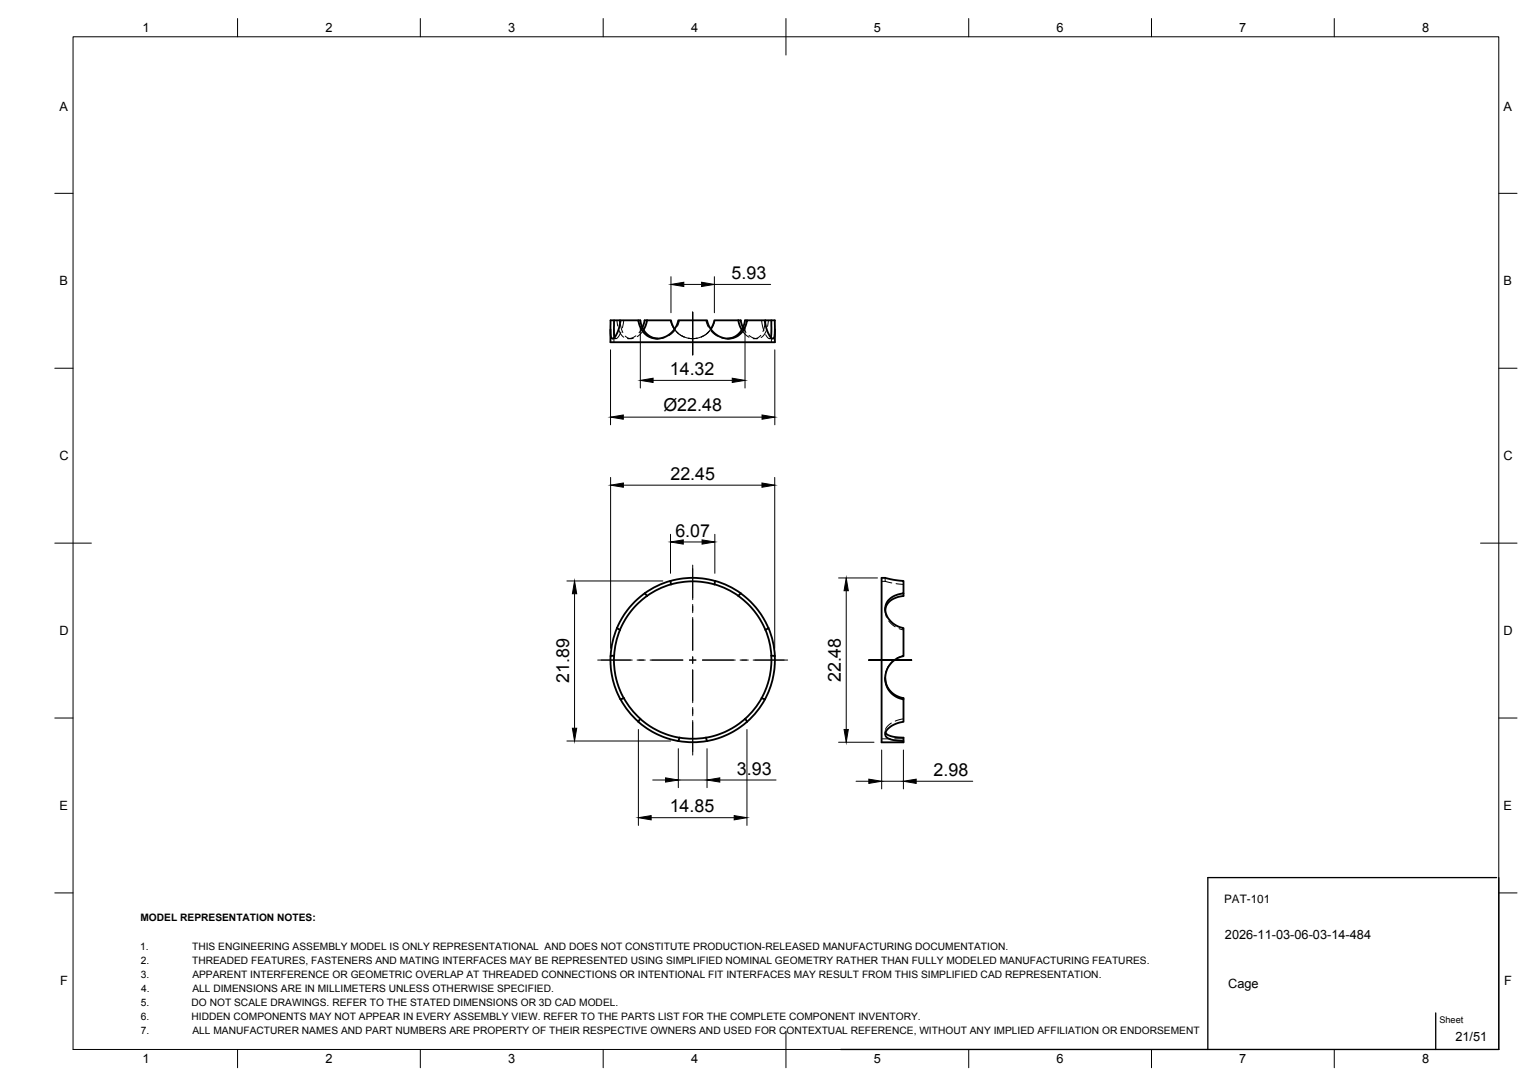
ISO-10303-21;
HEADER;
/* Generated by software containing ST-Developer
 * from STEP Tools, Inc. (www.steptools.com) 
 */

FILE_DESCRIPTION(
/* description */ ('Spur gear reduction stage 2-1 on bearing plates'),
/* implementation_level */ '2;1');

FILE_NAME(
/* name */ 'Cage.step',
/* time_stamp */ '2026-10-28T03:22:07-07:00',
/* author */ (''),
/* organization */ (''),
/* preprocessor_version */ 'ST-DEVELOPER v20.2',
/* originating_system */ 'Autodesk Translation Framework v15.17.0.0',
/* authorisation */ '');

FILE_SCHEMA (('AUTOMOTIVE_DESIGN { 1 0 10303 214 3 1 1 }'));
ENDSEC;

DATA;
#10=MECHANICAL_DESIGN_GEOMETRIC_PRESENTATION_REPRESENTATION('',(#969),#53909);
#667=B_SPLINE_CURVE_WITH_KNOTS('',3,(#16802,#16803,#16804,#16805,#16806,
#16807,#16808,#16809,#16810,#16811,#16812,#16813,#16814,#16815,#16816,#16817,
#16818,#16819,#16820,#16821,#16822,#16823),.UNSPECIFIED.,.F.,.F.,(4,2,2,
2,2,2,2,2,2,2,4),(0.0591825211272536,0.157966726598481,0.236950089897721,
0.315933453196962,0.391576304923761,0.46721915665056,0.54286200837736,0.618504860104159,
0.697488223403399,0.77647158670264,0.875255792173867),.UNSPECIFIED.);
#668=B_SPLINE_CURVE_WITH_KNOTS('',3,(#16827,#16828,#16829,#16830,#16831,
#16832,#16833,#16834,#16835,#16836,#16837,#16838,#16839,#16840,#16841,#16842,
#16843,#16844,#16845,#16846,#16847,#16848),.UNSPECIFIED.,.F.,.F.,(4,2,2,
2,2,2,2,2,2,2,4),(0.0581119756758434,0.106553146291161,0.213106292582322,
0.30849933801665,0.386091982889075,0.4636846277615,0.541277272633925,0.61886991750635,
0.714262962940678,0.820816109231839,0.869257279847157),.UNSPECIFIED.);
#669=B_SPLINE_CURVE_WITH_KNOTS('',3,(#16854,#16855,#16856,#16857,#16858,
#16859,#16860,#16861,#16862,#16863,#16864,#16865,#16866,#16867,#16868,#16869,
#16870,#16871,#16872,#16873,#16874,#16875),.UNSPECIFIED.,.F.,.F.,(4,2,2,
2,2,2,2,2,2,2,4),(0.0581119756758434,0.106553146291161,0.213106292582322,
0.30849933801665,0.386091982889075,0.4636846277615,0.541277272633925,0.61886991750635,
0.714262962940679,0.820816109231839,0.869257279847157),.UNSPECIFIED.);
#670=B_SPLINE_CURVE_WITH_KNOTS('',3,(#16879,#16880,#16881,#16882,#16883,
#16884,#16885,#16886,#16887,#16888,#16889,#16890,#16891,#16892,#16893,#16894,
#16895,#16896,#16897,#16898,#16899,#16900),.UNSPECIFIED.,.F.,.F.,(4,2,2,
2,2,2,2,2,2,2,4),(0.0581119756758433,0.106553146291161,0.213106292582322,
0.308499338016649,0.386091982889075,0.4636846277615,0.541277272633925,0.61886991750635,
0.714262962940678,0.820816109231839,0.869257279847157),.UNSPECIFIED.);
#671=B_SPLINE_CURVE_WITH_KNOTS('',3,(#16909,#16910,#16911,#16912,#16913,
#16914,#16915,#16916,#16917,#16918,#16919,#16920,#16921,#16922,#16923,#16924,
#16925,#16926,#16927,#16928,#16929,#16930),.UNSPECIFIED.,.F.,.F.,(4,2,2,
2,2,2,2,2,2,2,4),(0.0581119756758433,0.106553146291161,0.213106292582322,
0.30849933801665,0.386091982889075,0.4636846277615,0.541277272633925,0.61886991750635,
0.714262962940678,0.820816109231839,0.869257279847157),.UNSPECIFIED.);
#672=B_SPLINE_CURVE_WITH_KNOTS('',3,(#16934,#16935,#16936,#16937,#16938,
#16939,#16940,#16941,#16942,#16943,#16944,#16945,#16946,#16947,#16948,#16949,
#16950,#16951,#16952,#16953,#16954,#16955),.UNSPECIFIED.,.F.,.F.,(4,2,2,
2,2,2,2,2,2,2,4),(0.0581119756758434,0.106553146291161,0.213106292582322,
0.30849933801665,0.386091982889075,0.4636846277615,0.541277272633925,0.61886991750635,
0.714262962940678,0.820816109231839,0.869257279847157),.UNSPECIFIED.);
#673=B_SPLINE_CURVE_WITH_KNOTS('',3,(#16959,#16960,#16961,#16962,#16963,
#16964,#16965,#16966,#16967,#16968,#16969,#16970,#16971,#16972,#16973,#16974,
#16975,#16976,#16977,#16978,#16979,#16980),.UNSPECIFIED.,.F.,.F.,(4,2,2,
2,2,2,2,2,2,2,4),(0.0581119756758434,0.106553146291161,0.213106292582322,
0.30849933801665,0.386091982889075,0.4636846277615,0.541277272633925,0.61886991750635,
0.714262962940678,0.820816109231839,0.869257279847157),.UNSPECIFIED.);
#674=B_SPLINE_CURVE_WITH_KNOTS('',3,(#16984,#16985,#16986,#16987,#16988,
#16989,#16990,#16991,#16992,#16993,#16994,#16995,#16996,#16997,#16998,#16999,
#17000,#17001,#17002,#17003,#17004,#17005),.UNSPECIFIED.,.F.,.F.,(4,2,2,
2,2,2,2,2,2,2,4),(0.0581119756758433,0.106553146291161,0.213106292582322,
0.30849933801665,0.386091982889075,0.4636846277615,0.541277272633925,0.61886991750635,
0.714262962940678,0.820816109231839,0.869257279847157),.UNSPECIFIED.);
#675=B_SPLINE_CURVE_WITH_KNOTS('',3,(#17013,#17014,#17015,#17016,#17017,
#17018,#17019,#17020,#17021,#17022,#17023,#17024,#17025,#17026,#17027,#17028,
#17029,#17030,#17031,#17032,#17033,#17034),.UNSPECIFIED.,.F.,.F.,(4,2,2,
2,2,2,2,2,2,2,4),(0.0591825211272536,0.157966726598481,0.236950089897721,
0.315933453196962,0.391576304923761,0.467219156650561,0.54286200837736,
0.618504860104159,0.697488223403399,0.77647158670264,0.875255792173867),
 .UNSPECIFIED.);
#676=B_SPLINE_CURVE_WITH_KNOTS('',3,(#17042,#17043,#17044,#17045,#17046,
#17047,#17048,#17049,#17050,#17051,#17052,#17053,#17054,#17055,#17056,#17057,
#17058,#17059,#17060,#17061,#17062,#17063),.UNSPECIFIED.,.F.,.F.,(4,2,2,
2,2,2,2,2,2,2,4),(0.0591825211272536,0.157966726598481,0.236950089897722,
0.315933453196962,0.391576304923761,0.467219156650561,0.54286200837736,
0.618504860104159,0.697488223403399,0.77647158670264,0.875255792173867),
 .UNSPECIFIED.);
#677=B_SPLINE_CURVE_WITH_KNOTS('',3,(#17073,#17074,#17075,#17076,#17077,
#17078,#17079,#17080,#17081,#17082,#17083,#17084,#17085,#17086,#17087,#17088,
#17089,#17090,#17091,#17092,#17093,#17094),.UNSPECIFIED.,.F.,.F.,(4,2,2,
2,2,2,2,2,2,2,4),(0.0591825211272536,0.157966726598481,0.236950089897721,
0.315933453196962,0.391576304923761,0.46721915665056,0.54286200837736,0.618504860104159,
0.697488223403399,0.77647158670264,0.875255792173867),.UNSPECIFIED.);
#678=B_SPLINE_CURVE_WITH_KNOTS('',3,(#17102,#17103,#17104,#17105,#17106,
#17107,#17108,#17109,#17110,#17111,#17112,#17113,#17114,#17115,#17116,#17117,
#17118,#17119,#17120,#17121,#17122,#17123),.UNSPECIFIED.,.F.,.F.,(4,2,2,
2,2,2,2,2,2,2,4),(0.0591825211272536,0.157966726598481,0.236950089897721,
0.315933453196962,0.391576304923761,0.46721915665056,0.542862008377359,
0.618504860104159,0.697488223403399,0.776471586702639,0.875255792173867),
 .UNSPECIFIED.);
#679=B_SPLINE_CURVE_WITH_KNOTS('',3,(#17131,#17132,#17133,#17134,#17135,
#17136,#17137,#17138,#17139,#17140,#17141,#17142,#17143,#17144,#17145,#17146,
#17147,#17148,#17149,#17150,#17151,#17152),.UNSPECIFIED.,.F.,.F.,(4,2,2,
2,2,2,2,2,2,2,4),(0.0591825211272536,0.157966726598481,0.236950089897721,
0.315933453196962,0.391576304923761,0.46721915665056,0.54286200837736,0.618504860104159,
0.697488223403399,0.77647158670264,0.875255792173867),.UNSPECIFIED.);
#680=B_SPLINE_CURVE_WITH_KNOTS('',3,(#17161,#17162,#17163,#17164,#17165,
#17166,#17167,#17168,#17169,#17170,#17171,#17172,#17173,#17174,#17175,#17176,
#17177,#17178,#17179,#17180,#17181,#17182),.UNSPECIFIED.,.F.,.F.,(4,2,2,
2,2,2,2,2,2,2,4),(0.0591825211272536,0.157966726598481,0.236950089897721,
0.315933453196962,0.391576304923761,0.46721915665056,0.542862008377359,
0.618504860104159,0.697488223403399,0.776471586702639,0.875255792173867),
 .UNSPECIFIED.);
#802=SPHERICAL_SURFACE('',#12210,0.309556);
#803=SPHERICAL_SURFACE('',#12226,0.309556);
#804=SPHERICAL_SURFACE('',#12231,0.309556);
#805=SPHERICAL_SURFACE('',#12237,0.309556);
#806=SPHERICAL_SURFACE('',#12242,0.309556);
#807=SPHERICAL_SURFACE('',#12247,0.309556);
#808=SPHERICAL_SURFACE('',#12255,0.309556);
#877=SHAPE_REPRESENTATION_RELATIONSHIP('SRR','None',#54105,#920);
#920=ADVANCED_BREP_SHAPE_REPRESENTATION('',(#1025),#53879);
#969=STYLED_ITEM('',(#54397),#1025);
#1025=MANIFOLD_SOLID_BREP('Continuous crown cage',#11295);
#1182=FACE_BOUND('',#2476,.T.);
#1318=PLANE('',#12223);
#1319=PLANE('',#12228);
#1320=PLANE('',#12233);
#1321=PLANE('',#12239);
#1322=PLANE('',#12244);
#1323=PLANE('',#12253);
#1324=PLANE('',#12257);
#1325=PLANE('',#12258);
#1690=FACE_OUTER_BOUND('',#2460,.T.);
#1691=FACE_OUTER_BOUND('',#2461,.T.);
#1692=FACE_OUTER_BOUND('',#2462,.T.);
#1693=FACE_OUTER_BOUND('',#2463,.T.);
#1694=FACE_OUTER_BOUND('',#2464,.T.);
#1695=FACE_OUTER_BOUND('',#2465,.T.);
#1696=FACE_OUTER_BOUND('',#2466,.T.);
#1697=FACE_OUTER_BOUND('',#2467,.T.);
#1698=FACE_OUTER_BOUND('',#2468,.T.);
#1699=FACE_OUTER_BOUND('',#2469,.T.);
#1700=FACE_OUTER_BOUND('',#2470,.T.);
#1701=FACE_OUTER_BOUND('',#2471,.T.);
#1702=FACE_OUTER_BOUND('',#2472,.T.);
#1703=FACE_OUTER_BOUND('',#2473,.T.);
#1704=FACE_OUTER_BOUND('',#2474,.T.);
#1705=FACE_OUTER_BOUND('',#2475,.T.);
#1706=FACE_OUTER_BOUND('',#2477,.T.);
#2460=EDGE_LOOP('',(#8086,#8087,#8088,#8089));
#2461=EDGE_LOOP('',(#8090,#8091,#8092,#8093,#8094,#8095,#8096,#8097,#8098,
#8099,#8100,#8101,#8102,#8103,#8104,#8105,#8106,#8107));
#2462=EDGE_LOOP('',(#8108,#8109,#8110,#8111));
#2463=EDGE_LOOP('',(#8112,#8113,#8114,#8115));
#2464=EDGE_LOOP('',(#8116,#8117,#8118,#8119));
#2465=EDGE_LOOP('',(#8120,#8121,#8122,#8123));
#2466=EDGE_LOOP('',(#8124,#8125,#8126,#8127,#8128,#8129));
#2467=EDGE_LOOP('',(#8130,#8131,#8132,#8133));
#2468=EDGE_LOOP('',(#8134,#8135,#8136,#8137));
#2469=EDGE_LOOP('',(#8138,#8139,#8140,#8141));
#2470=EDGE_LOOP('',(#8142,#8143,#8144,#8145));
#2471=EDGE_LOOP('',(#8146,#8147,#8148,#8149));
#2472=EDGE_LOOP('',(#8150,#8151,#8152,#8153,#8154,#8155,#8156,#8157,#8158,
#8159,#8160,#8161,#8162,#8163,#8164,#8165,#8166,#8167));
#2473=EDGE_LOOP('',(#8168,#8169,#8170,#8171));
#2474=EDGE_LOOP('',(#8172,#8173,#8174,#8175));
#2475=EDGE_LOOP('',(#8176));
#2476=EDGE_LOOP('',(#8177));
#2477=EDGE_LOOP('',(#8178,#8179,#8180,#8181));
#3147=LINE('',#16904,#3788);
#3148=LINE('',#17157,#3789);
#3788=VECTOR('',#13974,1.123812);
#3789=VECTOR('',#14043,1.076188);
#4456=CIRCLE('',#12211,0.303778037777585);
#4457=CIRCLE('',#12212,0.303778037777585);
#4458=CIRCLE('',#12214,1.123812);
#4459=CIRCLE('',#12215,1.123812);
#4460=CIRCLE('',#12216,1.123812);
#4461=CIRCLE('',#12217,1.123812);
#4462=CIRCLE('',#12218,1.123812);
#4463=CIRCLE('',#12219,1.123812);
#4464=CIRCLE('',#12220,1.123812);
#4465=CIRCLE('',#12221,1.123812);
#4466=CIRCLE('',#12222,1.123812);
#4467=CIRCLE('',#12224,1.076188);
#4468=CIRCLE('',#12225,0.303778037777585);
#4469=CIRCLE('',#12227,0.303778037777585);
#4470=CIRCLE('',#12229,1.076188);
#4471=CIRCLE('',#12230,0.303778037777585);
#4472=CIRCLE('',#12232,0.303778037777585);
#4473=CIRCLE('',#12234,1.076188);
#4474=CIRCLE('',#12235,1.076188);
#4475=CIRCLE('',#12236,0.303778037777585);
#4476=CIRCLE('',#12238,0.303778037777585);
#4477=CIRCLE('',#12240,1.076188);
#4478=CIRCLE('',#12241,0.303778037777585);
#4479=CIRCLE('',#12243,0.303778037777585);
#4480=CIRCLE('',#12245,1.076188);
#4481=CIRCLE('',#12246,0.303778037777585);
#4482=CIRCLE('',#12248,0.303778037777585);
#4483=CIRCLE('',#12250,1.076188);
#4484=CIRCLE('',#12251,1.076188);
#4485=CIRCLE('',#12252,1.076188);
#4486=CIRCLE('',#12254,0.303778037777585);
#4487=CIRCLE('',#12256,0.303778037777585);
#5034=VERTEX_POINT('',#16800);
#5035=VERTEX_POINT('',#16801);
#5036=VERTEX_POINT('',#16824);
#5037=VERTEX_POINT('',#16826);
#5038=VERTEX_POINT('',#16851);
#5039=VERTEX_POINT('',#16853);
#5040=VERTEX_POINT('',#16876);
#5041=VERTEX_POINT('',#16878);
#5042=VERTEX_POINT('',#16901);
#5043=VERTEX_POINT('',#16903);
#5044=VERTEX_POINT('',#16906);
#5045=VERTEX_POINT('',#16908);
#5046=VERTEX_POINT('',#16931);
#5047=VERTEX_POINT('',#16933);
#5048=VERTEX_POINT('',#16956);
#5049=VERTEX_POINT('',#16958);
#5050=VERTEX_POINT('',#16981);
#5051=VERTEX_POINT('',#16983);
#5052=VERTEX_POINT('',#17008);
#5053=VERTEX_POINT('',#17012);
#5054=VERTEX_POINT('',#17037);
#5055=VERTEX_POINT('',#17041);
#5056=VERTEX_POINT('',#17066);
#5057=VERTEX_POINT('',#17068);
#5058=VERTEX_POINT('',#17072);
#5059=VERTEX_POINT('',#17097);
#5060=VERTEX_POINT('',#17101);
#5061=VERTEX_POINT('',#17126);
#5062=VERTEX_POINT('',#17130);
#5063=VERTEX_POINT('',#17155);
#5064=VERTEX_POINT('',#17158);
#5065=VERTEX_POINT('',#17160);
#6185=EDGE_CURVE('',#5034,#5035,#667,.T.);
#6186=EDGE_CURVE('',#5036,#5034,#4456,.T.);
#6187=EDGE_CURVE('',#5037,#5036,#668,.T.);
#6188=EDGE_CURVE('',#5035,#5037,#4457,.T.);
#6189=EDGE_CURVE('',#5038,#5036,#4458,.T.);
#6190=EDGE_CURVE('',#5038,#5039,#669,.T.);
#6191=EDGE_CURVE('',#5040,#5039,#4459,.T.);
#6192=EDGE_CURVE('',#5040,#5041,#670,.T.);
#6193=EDGE_CURVE('',#5042,#5041,#4460,.T.);
#6194=EDGE_CURVE('',#5042,#5043,#3147,.T.);
#6195=EDGE_CURVE('',#5043,#5043,#4461,.T.);
#6196=EDGE_CURVE('',#5044,#5042,#4462,.T.);
#6197=EDGE_CURVE('',#5044,#5045,#671,.T.);
#6198=EDGE_CURVE('',#5046,#5045,#4463,.T.);
#6199=EDGE_CURVE('',#5046,#5047,#672,.T.);
#6200=EDGE_CURVE('',#5048,#5047,#4464,.T.);
#6201=EDGE_CURVE('',#5048,#5049,#673,.T.);
#6202=EDGE_CURVE('',#5050,#5049,#4465,.T.);
#6203=EDGE_CURVE('',#5050,#5051,#674,.T.);
#6204=EDGE_CURVE('',#5037,#5051,#4466,.T.);
#6205=EDGE_CURVE('',#5034,#5052,#4467,.T.);
#6206=EDGE_CURVE('',#5052,#5038,#4468,.T.);
#6207=EDGE_CURVE('',#5053,#5052,#675,.T.);
#6208=EDGE_CURVE('',#5039,#5053,#4469,.T.);
#6209=EDGE_CURVE('',#5053,#5054,#4470,.T.);
#6210=EDGE_CURVE('',#5054,#5040,#4471,.T.);
#6211=EDGE_CURVE('',#5055,#5054,#676,.T.);
#6212=EDGE_CURVE('',#5041,#5055,#4472,.T.);
#6213=EDGE_CURVE('',#5055,#5056,#4473,.T.);
#6214=EDGE_CURVE('',#5056,#5057,#4474,.T.);
#6215=EDGE_CURVE('',#5057,#5044,#4475,.T.);
#6216=EDGE_CURVE('',#5058,#5057,#677,.T.);
#6217=EDGE_CURVE('',#5045,#5058,#4476,.T.);
#6218=EDGE_CURVE('',#5058,#5059,#4477,.T.);
#6219=EDGE_CURVE('',#5059,#5046,#4478,.T.);
#6220=EDGE_CURVE('',#5060,#5059,#678,.T.);
#6221=EDGE_CURVE('',#5047,#5060,#4479,.T.);
#6222=EDGE_CURVE('',#5060,#5061,#4480,.T.);
#6223=EDGE_CURVE('',#5061,#5048,#4481,.T.);
#6224=EDGE_CURVE('',#5062,#5061,#679,.T.);
#6225=EDGE_CURVE('',#5049,#5062,#4482,.T.);
#6226=EDGE_CURVE('',#5063,#5063,#4483,.T.);
#6227=EDGE_CURVE('',#5063,#5056,#3148,.T.);
#6228=EDGE_CURVE('',#5064,#5035,#4484,.T.);
#6229=EDGE_CURVE('',#5064,#5065,#680,.T.);
#6230=EDGE_CURVE('',#5062,#5065,#4485,.T.);
#6231=EDGE_CURVE('',#5051,#5064,#4486,.T.);
#6232=EDGE_CURVE('',#5065,#5050,#4487,.T.);
#8086=ORIENTED_EDGE('',*,*,#6185,.F.);
#8087=ORIENTED_EDGE('',*,*,#6186,.F.);
#8088=ORIENTED_EDGE('',*,*,#6187,.F.);
#8089=ORIENTED_EDGE('',*,*,#6188,.F.);
#8090=ORIENTED_EDGE('',*,*,#6187,.T.);
#8091=ORIENTED_EDGE('',*,*,#6189,.F.);
#8092=ORIENTED_EDGE('',*,*,#6190,.T.);
#8093=ORIENTED_EDGE('',*,*,#6191,.F.);
#8094=ORIENTED_EDGE('',*,*,#6192,.T.);
#8095=ORIENTED_EDGE('',*,*,#6193,.F.);
#8096=ORIENTED_EDGE('',*,*,#6194,.T.);
#8097=ORIENTED_EDGE('',*,*,#6195,.F.);
#8098=ORIENTED_EDGE('',*,*,#6194,.F.);
#8099=ORIENTED_EDGE('',*,*,#6196,.F.);
#8100=ORIENTED_EDGE('',*,*,#6197,.T.);
#8101=ORIENTED_EDGE('',*,*,#6198,.F.);
#8102=ORIENTED_EDGE('',*,*,#6199,.T.);
#8103=ORIENTED_EDGE('',*,*,#6200,.F.);
#8104=ORIENTED_EDGE('',*,*,#6201,.T.);
#8105=ORIENTED_EDGE('',*,*,#6202,.F.);
#8106=ORIENTED_EDGE('',*,*,#6203,.T.);
#8107=ORIENTED_EDGE('',*,*,#6204,.F.);
#8108=ORIENTED_EDGE('',*,*,#6186,.T.);
#8109=ORIENTED_EDGE('',*,*,#6205,.T.);
#8110=ORIENTED_EDGE('',*,*,#6206,.T.);
#8111=ORIENTED_EDGE('',*,*,#6189,.T.);
#8112=ORIENTED_EDGE('',*,*,#6207,.F.);
#8113=ORIENTED_EDGE('',*,*,#6208,.F.);
#8114=ORIENTED_EDGE('',*,*,#6190,.F.);
#8115=ORIENTED_EDGE('',*,*,#6206,.F.);
#8116=ORIENTED_EDGE('',*,*,#6208,.T.);
#8117=ORIENTED_EDGE('',*,*,#6209,.T.);
#8118=ORIENTED_EDGE('',*,*,#6210,.T.);
#8119=ORIENTED_EDGE('',*,*,#6191,.T.);
#8120=ORIENTED_EDGE('',*,*,#6211,.F.);
#8121=ORIENTED_EDGE('',*,*,#6212,.F.);
#8122=ORIENTED_EDGE('',*,*,#6192,.F.);
#8123=ORIENTED_EDGE('',*,*,#6210,.F.);
#8124=ORIENTED_EDGE('',*,*,#6212,.T.);
#8125=ORIENTED_EDGE('',*,*,#6213,.T.);
#8126=ORIENTED_EDGE('',*,*,#6214,.T.);
#8127=ORIENTED_EDGE('',*,*,#6215,.T.);
#8128=ORIENTED_EDGE('',*,*,#6196,.T.);
#8129=ORIENTED_EDGE('',*,*,#6193,.T.);
#8130=ORIENTED_EDGE('',*,*,#6216,.F.);
#8131=ORIENTED_EDGE('',*,*,#6217,.F.);
#8132=ORIENTED_EDGE('',*,*,#6197,.F.);
#8133=ORIENTED_EDGE('',*,*,#6215,.F.);
#8134=ORIENTED_EDGE('',*,*,#6217,.T.);
#8135=ORIENTED_EDGE('',*,*,#6218,.T.);
#8136=ORIENTED_EDGE('',*,*,#6219,.T.);
#8137=ORIENTED_EDGE('',*,*,#6198,.T.);
#8138=ORIENTED_EDGE('',*,*,#6220,.F.);
#8139=ORIENTED_EDGE('',*,*,#6221,.F.);
#8140=ORIENTED_EDGE('',*,*,#6199,.F.);
#8141=ORIENTED_EDGE('',*,*,#6219,.F.);
#8142=ORIENTED_EDGE('',*,*,#6221,.T.);
#8143=ORIENTED_EDGE('',*,*,#6222,.T.);
#8144=ORIENTED_EDGE('',*,*,#6223,.T.);
#8145=ORIENTED_EDGE('',*,*,#6200,.T.);
#8146=ORIENTED_EDGE('',*,*,#6201,.F.);
#8147=ORIENTED_EDGE('',*,*,#6223,.F.);
#8148=ORIENTED_EDGE('',*,*,#6224,.F.);
#8149=ORIENTED_EDGE('',*,*,#6225,.F.);
#8150=ORIENTED_EDGE('',*,*,#6226,.F.);
#8151=ORIENTED_EDGE('',*,*,#6227,.T.);
#8152=ORIENTED_EDGE('',*,*,#6213,.F.);
#8153=ORIENTED_EDGE('',*,*,#6211,.T.);
#8154=ORIENTED_EDGE('',*,*,#6209,.F.);
#8155=ORIENTED_EDGE('',*,*,#6207,.T.);
#8156=ORIENTED_EDGE('',*,*,#6205,.F.);
#8157=ORIENTED_EDGE('',*,*,#6185,.T.);
#8158=ORIENTED_EDGE('',*,*,#6228,.F.);
#8159=ORIENTED_EDGE('',*,*,#6229,.T.);
#8160=ORIENTED_EDGE('',*,*,#6230,.F.);
#8161=ORIENTED_EDGE('',*,*,#6224,.T.);
#8162=ORIENTED_EDGE('',*,*,#6222,.F.);
#8163=ORIENTED_EDGE('',*,*,#6220,.T.);
#8164=ORIENTED_EDGE('',*,*,#6218,.F.);
#8165=ORIENTED_EDGE('',*,*,#6216,.T.);
#8166=ORIENTED_EDGE('',*,*,#6214,.F.);
#8167=ORIENTED_EDGE('',*,*,#6227,.F.);
#8168=ORIENTED_EDGE('',*,*,#6188,.T.);
#8169=ORIENTED_EDGE('',*,*,#6204,.T.);
#8170=ORIENTED_EDGE('',*,*,#6231,.T.);
#8171=ORIENTED_EDGE('',*,*,#6228,.T.);
#8172=ORIENTED_EDGE('',*,*,#6203,.F.);
#8173=ORIENTED_EDGE('',*,*,#6232,.F.);
#8174=ORIENTED_EDGE('',*,*,#6229,.F.);
#8175=ORIENTED_EDGE('',*,*,#6231,.F.);
#8176=ORIENTED_EDGE('',*,*,#6195,.T.);
#8177=ORIENTED_EDGE('',*,*,#6226,.T.);
#8178=ORIENTED_EDGE('',*,*,#6225,.T.);
#8179=ORIENTED_EDGE('',*,*,#6230,.T.);
#8180=ORIENTED_EDGE('',*,*,#6232,.T.);
#8181=ORIENTED_EDGE('',*,*,#6202,.T.);
#10506=CYLINDRICAL_SURFACE('',#12213,1.123812);
#10507=CYLINDRICAL_SURFACE('',#12249,1.076188);
#10810=ADVANCED_FACE('',(#1690),#802,.F.);
#10811=ADVANCED_FACE('',(#1691),#10506,.T.);
#10812=ADVANCED_FACE('',(#1692),#1318,.T.);
#10813=ADVANCED_FACE('',(#1693),#803,.F.);
#10814=ADVANCED_FACE('',(#1694),#1319,.T.);
#10815=ADVANCED_FACE('',(#1695),#804,.F.);
#10816=ADVANCED_FACE('',(#1696),#1320,.T.);
#10817=ADVANCED_FACE('',(#1697),#805,.F.);
#10818=ADVANCED_FACE('',(#1698),#1321,.T.);
#10819=ADVANCED_FACE('',(#1699),#806,.F.);
#10820=ADVANCED_FACE('',(#1700),#1322,.T.);
#10821=ADVANCED_FACE('',(#1701),#807,.F.);
#10822=ADVANCED_FACE('',(#1702),#10507,.F.);
#10823=ADVANCED_FACE('',(#1703),#1323,.T.);
#10824=ADVANCED_FACE('',(#1704),#808,.F.);
#10825=ADVANCED_FACE('',(#1705,#1182),#1324,.T.);
#10826=ADVANCED_FACE('',(#1706),#1325,.T.);
#11295=CLOSED_SHELL('',(#10810,#10811,#10812,#10813,#10814,#10815,#10816,
#10817,#10818,#10819,#10820,#10821,#10822,#10823,#10824,#10825,#10826));
#12209=AXIS2_PLACEMENT_3D('',#16798,#13958,#13959);
#12210=AXIS2_PLACEMENT_3D('',#16799,#13960,#13961);
#12211=AXIS2_PLACEMENT_3D('',#16825,#13962,#13963);
#12212=AXIS2_PLACEMENT_3D('',#16849,#13964,#13965);
#12213=AXIS2_PLACEMENT_3D('',#16850,#13966,#13967);
#12214=AXIS2_PLACEMENT_3D('',#16852,#13968,#13969);
#12215=AXIS2_PLACEMENT_3D('',#16877,#13970,#13971);
#12216=AXIS2_PLACEMENT_3D('',#16902,#13972,#13973);
#12217=AXIS2_PLACEMENT_3D('',#16905,#13975,#13976);
#12218=AXIS2_PLACEMENT_3D('',#16907,#13977,#13978);
#12219=AXIS2_PLACEMENT_3D('',#16932,#13979,#13980);
#12220=AXIS2_PLACEMENT_3D('',#16957,#13981,#13982);
#12221=AXIS2_PLACEMENT_3D('',#16982,#13983,#13984);
#12222=AXIS2_PLACEMENT_3D('',#17006,#13985,#13986);
#12223=AXIS2_PLACEMENT_3D('',#17007,#13987,#13988);
#12224=AXIS2_PLACEMENT_3D('',#17009,#13989,#13990);
#12225=AXIS2_PLACEMENT_3D('',#17010,#13991,#13992);
#12226=AXIS2_PLACEMENT_3D('',#17011,#13993,#13994);
#12227=AXIS2_PLACEMENT_3D('',#17035,#13995,#13996);
#12228=AXIS2_PLACEMENT_3D('',#17036,#13997,#13998);
#12229=AXIS2_PLACEMENT_3D('',#17038,#13999,#14000);
#12230=AXIS2_PLACEMENT_3D('',#17039,#14001,#14002);
#12231=AXIS2_PLACEMENT_3D('',#17040,#14003,#14004);
#12232=AXIS2_PLACEMENT_3D('',#17064,#14005,#14006);
#12233=AXIS2_PLACEMENT_3D('',#17065,#14007,#14008);
#12234=AXIS2_PLACEMENT_3D('',#17067,#14009,#14010);
#12235=AXIS2_PLACEMENT_3D('',#17069,#14011,#14012);
#12236=AXIS2_PLACEMENT_3D('',#17070,#14013,#14014);
#12237=AXIS2_PLACEMENT_3D('',#17071,#14015,#14016);
#12238=AXIS2_PLACEMENT_3D('',#17095,#14017,#14018);
#12239=AXIS2_PLACEMENT_3D('',#17096,#14019,#14020);
#12240=AXIS2_PLACEMENT_3D('',#17098,#14021,#14022);
#12241=AXIS2_PLACEMENT_3D('',#17099,#14023,#14024);
#12242=AXIS2_PLACEMENT_3D('',#17100,#14025,#14026);
#12243=AXIS2_PLACEMENT_3D('',#17124,#14027,#14028);
#12244=AXIS2_PLACEMENT_3D('',#17125,#14029,#14030);
#12245=AXIS2_PLACEMENT_3D('',#17127,#14031,#14032);
#12246=AXIS2_PLACEMENT_3D('',#17128,#14033,#14034);
#12247=AXIS2_PLACEMENT_3D('',#17129,#14035,#14036);
#12248=AXIS2_PLACEMENT_3D('',#17153,#14037,#14038);
#12249=AXIS2_PLACEMENT_3D('',#17154,#14039,#14040);
#12250=AXIS2_PLACEMENT_3D('',#17156,#14041,#14042);
#12251=AXIS2_PLACEMENT_3D('',#17159,#14044,#14045);
#12252=AXIS2_PLACEMENT_3D('',#17183,#14046,#14047);
#12253=AXIS2_PLACEMENT_3D('',#17184,#14048,#14049);
#12254=AXIS2_PLACEMENT_3D('',#17185,#14050,#14051);
#12255=AXIS2_PLACEMENT_3D('',#17186,#14052,#14053);
#12256=AXIS2_PLACEMENT_3D('',#17187,#14054,#14055);
#12257=AXIS2_PLACEMENT_3D('',#17188,#14056,#14057);
#12258=AXIS2_PLACEMENT_3D('',#17189,#14058,#14059);
#13958=DIRECTION('axis',(0.,0.,1.));
#13959=DIRECTION('refdir',(1.,0.,0.));
#13960=DIRECTION('center_axis',(0.,0.,1.));
#13961=DIRECTION('ref_axis',(1.,0.,0.));
#13962=DIRECTION('center_axis',(0.,-1.,0.));
#13963=DIRECTION('ref_axis',(0.,0.,-1.));
#13964=DIRECTION('center_axis',(0.,-1.,0.));
#13965=DIRECTION('ref_axis',(0.,0.,-1.));
#13966=DIRECTION('center_axis',(0.,1.,0.));
#13967=DIRECTION('ref_axis',(1.,0.,0.));
#13968=DIRECTION('center_axis',(0.,1.,0.));
#13969=DIRECTION('ref_axis',(1.,0.,0.));
#13970=DIRECTION('center_axis',(0.,1.,0.));
#13971=DIRECTION('ref_axis',(1.,0.,0.));
#13972=DIRECTION('center_axis',(0.,1.,0.));
#13973=DIRECTION('ref_axis',(1.,0.,0.));
#13974=DIRECTION('',(0.,-1.,0.));
#13975=DIRECTION('center_axis',(0.,-1.,0.));
#13976=DIRECTION('ref_axis',(1.,0.,0.));
#13977=DIRECTION('center_axis',(0.,1.,0.));
#13978=DIRECTION('ref_axis',(1.,0.,0.));
#13979=DIRECTION('center_axis',(0.,1.,0.));
#13980=DIRECTION('ref_axis',(1.,0.,0.));
#13981=DIRECTION('center_axis',(0.,1.,0.));
#13982=DIRECTION('ref_axis',(1.,0.,0.));
#13983=DIRECTION('center_axis',(0.,1.,0.));
#13984=DIRECTION('ref_axis',(1.,0.,0.));
#13985=DIRECTION('center_axis',(0.,1.,0.));
#13986=DIRECTION('ref_axis',(1.,0.,0.));
#13987=DIRECTION('center_axis',(0.,1.,0.));
#13988=DIRECTION('ref_axis',(1.,0.,0.));
#13989=DIRECTION('center_axis',(0.,-1.,0.));
#13990=DIRECTION('ref_axis',(1.,0.,0.));
#13991=DIRECTION('center_axis',(0.,-1.,0.));
#13992=DIRECTION('ref_axis',(0.,0.,-1.));
#13993=DIRECTION('center_axis',(8.96625347776458E-17,0.,1.));
#13994=DIRECTION('ref_axis',(1.,0.,0.));
#13995=DIRECTION('center_axis',(0.,-1.,0.));
#13996=DIRECTION('ref_axis',(0.,0.,-1.));
#13997=DIRECTION('center_axis',(0.,1.,0.));
#13998=DIRECTION('ref_axis',(1.,0.,0.));
#13999=DIRECTION('center_axis',(0.,-1.,0.));
#14000=DIRECTION('ref_axis',(1.,0.,0.));
#14001=DIRECTION('center_axis',(0.,-1.,0.));
#14002=DIRECTION('ref_axis',(0.,0.,-1.));
#14003=DIRECTION('center_axis',(0.,0.,1.));
#14004=DIRECTION('ref_axis',(1.,0.,0.));
#14005=DIRECTION('center_axis',(0.,-1.,0.));
#14006=DIRECTION('ref_axis',(0.,0.,-1.));
#14007=DIRECTION('center_axis',(0.,1.,0.));
#14008=DIRECTION('ref_axis',(1.,0.,0.));
#14009=DIRECTION('center_axis',(0.,-1.,0.));
#14010=DIRECTION('ref_axis',(1.,0.,0.));
#14011=DIRECTION('center_axis',(0.,-1.,0.));
#14012=DIRECTION('ref_axis',(1.,0.,0.));
#14013=DIRECTION('center_axis',(0.,-1.,0.));
#14014=DIRECTION('ref_axis',(0.,0.,-1.));
#14015=DIRECTION('center_axis',(0.,0.,1.));
#14016=DIRECTION('ref_axis',(1.,0.,0.));
#14017=DIRECTION('center_axis',(0.,-1.,0.));
#14018=DIRECTION('ref_axis',(0.,0.,-1.));
#14019=DIRECTION('center_axis',(0.,1.,0.));
#14020=DIRECTION('ref_axis',(1.,0.,0.));
#14021=DIRECTION('center_axis',(0.,-1.,0.));
#14022=DIRECTION('ref_axis',(1.,0.,0.));
#14023=DIRECTION('center_axis',(0.,-1.,0.));
#14024=DIRECTION('ref_axis',(0.,0.,-1.));
#14025=DIRECTION('center_axis',(8.96625347776458E-17,0.,1.));
#14026=DIRECTION('ref_axis',(1.,0.,0.));
#14027=DIRECTION('center_axis',(0.,-1.,0.));
#14028=DIRECTION('ref_axis',(0.,0.,-1.));
#14029=DIRECTION('center_axis',(0.,1.,0.));
#14030=DIRECTION('ref_axis',(1.,0.,0.));
#14031=DIRECTION('center_axis',(0.,-1.,0.));
#14032=DIRECTION('ref_axis',(1.,0.,0.));
#14033=DIRECTION('center_axis',(0.,-1.,0.));
#14034=DIRECTION('ref_axis',(0.,0.,-1.));
#14035=DIRECTION('center_axis',(0.,0.,1.));
#14036=DIRECTION('ref_axis',(1.,0.,0.));
#14037=DIRECTION('center_axis',(0.,-1.,0.));
#14038=DIRECTION('ref_axis',(0.,0.,-1.));
#14039=DIRECTION('center_axis',(0.,1.,0.));
#14040=DIRECTION('ref_axis',(1.,0.,0.));
#14041=DIRECTION('center_axis',(0.,1.,0.));
#14042=DIRECTION('ref_axis',(1.,0.,0.));
#14043=DIRECTION('',(0.,1.,0.));
#14044=DIRECTION('center_axis',(0.,-1.,0.));
#14045=DIRECTION('ref_axis',(1.,0.,0.));
#14046=DIRECTION('center_axis',(0.,-1.,0.));
#14047=DIRECTION('ref_axis',(1.,0.,0.));
#14048=DIRECTION('center_axis',(0.,1.,0.));
#14049=DIRECTION('ref_axis',(1.,0.,0.));
#14050=DIRECTION('center_axis',(0.,-1.,0.));
#14051=DIRECTION('ref_axis',(0.,0.,-1.));
#14052=DIRECTION('center_axis',(0.,0.,1.));
#14053=DIRECTION('ref_axis',(1.,0.,0.));
#14054=DIRECTION('center_axis',(0.,-1.,0.));
#14055=DIRECTION('ref_axis',(0.,0.,-1.));
#14056=DIRECTION('center_axis',(0.,-1.,0.));
#14057=DIRECTION('ref_axis',(-1.,0.,0.));
#14058=DIRECTION('center_axis',(0.,1.,0.));
#14059=DIRECTION('ref_axis',(1.,0.,0.));
#16798=CARTESIAN_POINT('',(0.,0.,0.));
#16799=CARTESIAN_POINT('Origin',(0.685838782044607,0.,0.860014630714833));
#16800=CARTESIAN_POINT('',(0.413083465285518,-0.05953,0.993751811093549));
#16801=CARTESIAN_POINT('',(0.876916659919095,-0.05953,0.623857181492959));
#16802=CARTESIAN_POINT('Ctrl Pts',(0.413083465285518,-0.05953,0.993751811093549));
#16803=CARTESIAN_POINT('Ctrl Pts',(0.419070565453383,-0.0925528133349865,
0.991263089003441));
#16804=CARTESIAN_POINT('Ctrl Pts',(0.430199341854858,-0.124911173756694,
0.986608710139579));
#16805=CARTESIAN_POINT('Ctrl Pts',(0.457978755888596,-0.177924977804098,
0.973971221090534));
#16806=CARTESIAN_POINT('Ctrl Pts',(0.473077587363685,-0.199697230012983,
0.966820759530997));
#16807=CARTESIAN_POINT('Ctrl Pts',(0.507057380724533,-0.237895043532788,
0.949440676105255));
#16808=CARTESIAN_POINT('Ctrl Pts',(0.525933334162555,-0.254319232363049,
0.939198248544428));
#16809=CARTESIAN_POINT('Ctrl Pts',(0.564362943424238,-0.28018331644634,
0.916597376014514));
#16810=CARTESIAN_POINT('Ctrl Pts',(0.585840553788742,-0.29104845371857,
0.903141581680914));
#16811=CARTESIAN_POINT('Ctrl Pts',(0.629305439856167,-0.30527573347708,
0.873412008702649));
#16812=CARTESIAN_POINT('Ctrl Pts',(0.651278921914856,-0.308638795020976,
0.857118508332695));
#16813=CARTESIAN_POINT('Ctrl Pts',(0.690705563850638,-0.308638795020976,
0.825676810575914));
#16814=CARTESIAN_POINT('Ctrl Pts',(0.711480111898423,-0.30527573347708,
0.807879894508811));
#16815=CARTESIAN_POINT('Ctrl Pts',(0.750136149454208,-0.29104845371857,
0.772120216227122));
#16816=CARTESIAN_POINT('Ctrl Pts',(0.768033796848072,-0.28018331644634,
0.754175290318038));
#16817=CARTESIAN_POINT('Ctrl Pts',(0.798619410861634,-0.254319232363049,
0.721738358858166));
#16818=CARTESIAN_POINT('Ctrl Pts',(0.812805334167529,-0.237895043532788,
0.705614819529209));
#16819=CARTESIAN_POINT('Ctrl Pts',(0.837310877969633,-0.199697230012983,
0.676354402927683));
#16820=CARTESIAN_POINT('Ctrl Pts',(0.847641868610495,-0.177924977804098,
0.663225258065736));
#16821=CARTESIAN_POINT('Ctrl Pts',(0.866144010579847,-0.124911173756694,
0.638954437806245));
#16822=CARTESIAN_POINT('Ctrl Pts',(0.873158080166742,-0.0925528133349865,
0.62914037979579));
#16823=CARTESIAN_POINT('Ctrl Pts',(0.876916659919095,-0.05953,0.623857181492959));
#16824=CARTESIAN_POINT('',(0.437601487681057,-0.05953,1.03511272300331));
#16825=CARTESIAN_POINT('Origin',(0.685838782044607,-0.05953,0.860014630714833));
#16826=CARTESIAN_POINT('',(0.911784794170997,-0.05953,0.656964154625313));
#16827=CARTESIAN_POINT('Ctrl Pts',(0.911784794170998,-0.0595300000000001,
0.656964154625312));
#16828=CARTESIAN_POINT('Ctrl Pts',(0.909827729890942,-0.0762225747374255,
0.659680317203144));
#16829=CARTESIAN_POINT('Ctrl Pts',(0.907004864562642,-0.0928409665394228,
0.663576540841106));
#16830=CARTESIAN_POINT('Ctrl Pts',(0.895234408667242,-0.144299303100741,
0.679480524217551));
#16831=CARTESIAN_POINT('Ctrl Pts',(0.882797231409153,-0.177024326825049,
0.695831250979106));
#16832=CARTESIAN_POINT('Ctrl Pts',(0.854332839576145,-0.227269801620064,
0.73042219438957));
#16833=CARTESIAN_POINT('Ctrl Pts',(0.834863020612702,-0.251265615809407,
0.752807465209441));
#16834=CARTESIAN_POINT('Ctrl Pts',(0.800439809856111,-0.279889827963178,
0.789147407129766));
#16835=CARTESIAN_POINT('Ctrl Pts',(0.781998747691871,-0.290879136862659,
0.80756613568454));
#16836=CARTESIAN_POINT('Ctrl Pts',(0.742239891936898,-0.305251990234487,
0.844254137480382));
#16837=CARTESIAN_POINT('Ctrl Pts',(0.720906778729541,-0.308638795020976,
0.862505527716294));
#16838=CARTESIAN_POINT('Ctrl Pts',(0.680463863683392,-0.308638795020976,
0.894757676234429));
#16839=CARTESIAN_POINT('Ctrl Pts',(0.657923009631182,-0.305251990234488,
0.91149460735272));
#16840=CARTESIAN_POINT('Ctrl Pts',(0.613307674922609,-0.290879136862659,
0.942092777160053));
#16841=CARTESIAN_POINT('Ctrl Pts',(0.591247219971725,-0.279889827963178,
0.955972930713954));
#16842=CARTESIAN_POINT('Ctrl Pts',(0.548158511259202,-0.251265615809407,
0.981446681891443));
#16843=CARTESIAN_POINT('Ctrl Pts',(0.522002043615455,-0.227269801620063,
0.995447160474328));
#16844=CARTESIAN_POINT('Ctrl Pts',(0.481944444320713,-0.177024326825049,
1.01550068154148));
#16845=CARTESIAN_POINT('Ctrl Pts',(0.463236132117164,-0.14429930310074,
1.0239876538093));
#16846=CARTESIAN_POINT('Ctrl Pts',(0.445111721969657,-0.0928409665394226,
1.03192403056628));
#16847=CARTESIAN_POINT('Ctrl Pts',(0.440685038163619,-0.0762225747374254,
1.03380912944435));
#16848=CARTESIAN_POINT('Ctrl Pts',(0.437601487681056,-0.05953,1.03511272300331));
#16849=CARTESIAN_POINT('Origin',(0.685838782044607,-0.05953,0.860014630714833));
#16850=CARTESIAN_POINT('Origin',(0.,-0.208355,0.));
#16851=CARTESIAN_POINT('',(0.0548532617164168,-0.05953,1.12247250791415));
#16852=CARTESIAN_POINT('Origin',(0.,-0.05953,0.));
#16853=CARTESIAN_POINT('',(-0.536443649899848,-0.05953,0.987512846410683));
#16854=CARTESIAN_POINT('Ctrl Pts',(0.0548532617164173,-0.0595300000000001,
1.12247250791414));
#16855=CARTESIAN_POINT('Ctrl Pts',(0.05150947068137,-0.0762225747374254,
1.12263591311425));
#16856=CARTESIAN_POINT('Ctrl Pts',(0.0467032526342597,-0.0928409665394227,
1.12285816383385));
#16857=CARTESIAN_POINT('Ctrl Pts',(0.0269302585198975,-0.144299303100741,
1.12357162229597));
#16858=CARTESIAN_POINT('Ctrl Pts',(0.006392292392153,-0.177024326825049,
1.12404235695137));
#16859=CARTESIAN_POINT('Ctrl Pts',(-0.0383992541984087,-0.227269801620063,
1.12335509974011));
#16860=CARTESIAN_POINT('Ctrl Pts',(-0.0680399972366993,-0.251265615809407,
1.12208997038458));
#16861=CARTESIAN_POINT('Ctrl Pts',(-0.117914228755037,-0.279889827963178,
1.1178344036749));
#16862=CARTESIAN_POINT('Ctrl Pts',(-0.14381238480104,-0.290879136862659,
1.11490049012186));
#16863=CARTESIAN_POINT('Ctrl Pts',(-0.19728546073067,-0.305251990234488,
1.10669035995599));
#16864=CARTESIAN_POINT('Ctrl Pts',(-0.224855950742601,-0.308638795020976,
1.10139101611326));
#16865=CARTESIAN_POINT('Ctrl Pts',(-0.275287440920027,-0.308638795020976,
1.0898803575765));
#16866=CARTESIAN_POINT('Ctrl Pts',(-0.302426893214945,-0.305251990234488,
1.08269251410343));
#16867=CARTESIAN_POINT('Ctrl Pts',(-0.35416671187353,-0.290879136862659,
1.06688848765783));
#16868=CARTESIAN_POINT('Ctrl Pts',(-0.3787731215897,-0.279889827963178,
1.05829506364875));
#16869=CARTESIAN_POINT('Ctrl Pts',(-0.425554672694338,-0.251265615809407,
1.04048957871266));
#16870=CARTESIAN_POINT('Ctrl Pts',(-0.452808978448581,-0.227269801620063,
1.02876878445619));
#16871=CARTESIAN_POINT('Ctrl Pts',(-0.493462957200432,-0.177024326825049,
1.0099536580922));
#16872=CARTESIAN_POINT('Ctrl Pts',(-0.511762781179148,-0.14429930310074,
1.00061845128527));
#16873=CARTESIAN_POINT('Ctrl Pts',(-0.529268075276157,-0.0928409665394226,
0.991396466802468));
#16874=CARTESIAN_POINT('Ctrl Pts',(-0.533501897135713,-0.0762225747374254,
0.989110885965947));
#16875=CARTESIAN_POINT('Ctrl Pts',(-0.536443649899848,-0.0595300000000001,
0.987512846410683));
#16876=CARTESIAN_POINT('',(-0.843383895613249,-0.05953,0.742736168477219));
#16877=CARTESIAN_POINT('Origin',(0.,-0.05953,0.));
#16878=CARTESIAN_POINT('',(-1.10653577764992,-0.05953,0.196295654879792));
#16879=CARTESIAN_POINT('Ctrl Pts',(-0.843383895613249,-0.0595300000000001,
0.742736168477219));
#16880=CARTESIAN_POINT('Ctrl Pts',(-0.84559647055299,-0.0762225747374255,
0.740223768851062));
#16881=CARTESIAN_POINT('Ctrl Pts',(-0.848766861100456,-0.0928409665394227,
0.736604687327351));
#16882=CARTESIAN_POINT('Ctrl Pts',(-0.861652925570091,-0.144299303100741,
0.721590372101268));
#16883=CARTESIAN_POINT('Ctrl Pts',(-0.87482617317514,-0.177024326825049,
0.705826641853758));
#16884=CARTESIAN_POINT('Ctrl Pts',(-0.902215926359523,-0.227269801620063,
0.670378702718353));
#16885=CARTESIAN_POINT('Ctrl Pts',(-0.919707509403859,-0.251265615809407,
0.646415841396062));
#16886=CARTESIAN_POINT('Ctrl Pts',(-0.947476448101718,-0.279889827963178,
0.604769294586516));
#16887=CARTESIAN_POINT('Ctrl Pts',(-0.961329858300736,-0.290879136862659,
0.582692035672022));
#16888=CARTESIAN_POINT('Ctrl Pts',(-0.988250837578047,-0.305251990234488,
0.535766169015486));
#16889=CARTESIAN_POINT('Ctrl Pts',(-1.00129756308006,-0.308638795020976,
0.510906605094603));
#16890=CARTESIAN_POINT('Ctrl Pts',(-1.02374168767024,-0.308638795020976,
0.46430090015576));
#16891=CARTESIAN_POINT('Ctrl Pts',(-1.03504317708586,-0.305251990234488,
0.438600874831839));
#16892=CARTESIAN_POINT('Ctrl Pts',(-1.05494634094458,-0.290879136862659,
0.388295406390235));
#16893=CARTESIAN_POINT('Ctrl Pts',(-1.06356957703048,-0.279889827963178,
0.363699428370917));
#16894=CARTESIAN_POINT('Ctrl Pts',(-1.0788165083757,-0.251265615809407,
0.316022600643821));
#16895=CARTESIAN_POINT('Ctrl Pts',(-1.08664560412098,-0.227269801620063,
0.287406530683752));
#16896=CARTESIAN_POINT('Ctrl Pts',(-1.09728268713976,-0.177024326825049,
0.243890930799337));
#16897=CARTESIAN_POINT('Ctrl Pts',(-1.10139388218929,-0.144299303100741,
0.22376314604679));
#16898=CARTESIAN_POINT('Ctrl Pts',(-1.10509821673782,-0.0928409665394227,
0.204327142733961));
#16899=CARTESIAN_POINT('Ctrl Pts',(-1.10595102243643,-0.0762225747374254,
0.199591971170104));
#16900=CARTESIAN_POINT('Ctrl Pts',(-1.10653577764992,-0.0595300000000001,
0.196295654879792));
#16901=CARTESIAN_POINT('',(-1.123812,-0.05953,1.37627276864339E-16));
#16902=CARTESIAN_POINT('Origin',(0.,-0.05953,0.));
#16903=CARTESIAN_POINT('',(-1.123812,-0.35718,1.37627276864339E-16));
#16904=CARTESIAN_POINT('',(-1.123812,-0.208355,1.37627276864339E-16));
#16905=CARTESIAN_POINT('Origin',(0.,-0.35718,0.));
#16906=CARTESIAN_POINT('',(-1.10653577764992,-0.05953,-0.196295654879793));
#16907=CARTESIAN_POINT('Origin',(0.,-0.05953,0.));
#16908=CARTESIAN_POINT('',(-0.843383895613249,-0.05953,-0.742736168477219));
#16909=CARTESIAN_POINT('Ctrl Pts',(-1.10653577764992,-0.0595300000000001,
-0.196295654879792));
#16910=CARTESIAN_POINT('Ctrl Pts',(-1.10595102243643,-0.0762225747374255,
-0.199591971170104));
#16911=CARTESIAN_POINT('Ctrl Pts',(-1.10509821673782,-0.0928409665394228,
-0.204327142733962));
#16912=CARTESIAN_POINT('Ctrl Pts',(-1.10139388218929,-0.144299303100741,
-0.22376314604679));
#16913=CARTESIAN_POINT('Ctrl Pts',(-1.09728268713976,-0.177024326825049,
-0.243890930799338));
#16914=CARTESIAN_POINT('Ctrl Pts',(-1.08664560412098,-0.227269801620063,
-0.287406530683753));
#16915=CARTESIAN_POINT('Ctrl Pts',(-1.0788165083757,-0.251265615809407,
-0.316022600643821));
#16916=CARTESIAN_POINT('Ctrl Pts',(-1.06356957703048,-0.279889827963178,
-0.363699428370918));
#16917=CARTESIAN_POINT('Ctrl Pts',(-1.05494634094458,-0.290879136862659,
-0.388295406390235));
#16918=CARTESIAN_POINT('Ctrl Pts',(-1.03504317708586,-0.305251990234488,
-0.438600874831839));
#16919=CARTESIAN_POINT('Ctrl Pts',(-1.02374168767024,-0.308638795020976,
-0.46430090015576));
#16920=CARTESIAN_POINT('Ctrl Pts',(-1.00129756308006,-0.308638795020976,
-0.510906605094603));
#16921=CARTESIAN_POINT('Ctrl Pts',(-0.988250837578047,-0.305251990234488,
-0.535766169015486));
#16922=CARTESIAN_POINT('Ctrl Pts',(-0.961329858300736,-0.290879136862659,
-0.582692035672022));
#16923=CARTESIAN_POINT('Ctrl Pts',(-0.947476448101718,-0.279889827963178,
-0.604769294586516));
#16924=CARTESIAN_POINT('Ctrl Pts',(-0.919707509403859,-0.251265615809407,
-0.646415841396062));
#16925=CARTESIAN_POINT('Ctrl Pts',(-0.902215926359523,-0.227269801620064,
-0.670378702718353));
#16926=CARTESIAN_POINT('Ctrl Pts',(-0.87482617317514,-0.177024326825049,
-0.705826641853758));
#16927=CARTESIAN_POINT('Ctrl Pts',(-0.861652925570091,-0.144299303100741,
-0.721590372101268));
#16928=CARTESIAN_POINT('Ctrl Pts',(-0.848766861100456,-0.0928409665394229,
-0.736604687327351));
#16929=CARTESIAN_POINT('Ctrl Pts',(-0.84559647055299,-0.0762225747374255,
-0.740223768851063));
#16930=CARTESIAN_POINT('Ctrl Pts',(-0.843383895613249,-0.0595300000000001,
-0.742736168477219));
#16931=CARTESIAN_POINT('',(-0.536443649899847,-0.05953,-0.987512846410683));
#16932=CARTESIAN_POINT('Origin',(0.,-0.05953,0.));
#16933=CARTESIAN_POINT('',(0.0548532617164172,-0.05953,-1.12247250791415));
#16934=CARTESIAN_POINT('Ctrl Pts',(-0.536443649899848,-0.0595300000000001,
-0.987512846410683));
#16935=CARTESIAN_POINT('Ctrl Pts',(-0.533501897135712,-0.0762225747374254,
-0.989110885965947));
#16936=CARTESIAN_POINT('Ctrl Pts',(-0.529268075276156,-0.0928409665394227,
-0.991396466802469));
#16937=CARTESIAN_POINT('Ctrl Pts',(-0.511762781179147,-0.144299303100741,
-1.00061845128527));
#16938=CARTESIAN_POINT('Ctrl Pts',(-0.493462957200432,-0.177024326825049,
-1.0099536580922));
#16939=CARTESIAN_POINT('Ctrl Pts',(-0.45280897844858,-0.227269801620063,
-1.02876878445619));
#16940=CARTESIAN_POINT('Ctrl Pts',(-0.425554672694337,-0.251265615809407,
-1.04048957871266));
#16941=CARTESIAN_POINT('Ctrl Pts',(-0.3787731215897,-0.279889827963178,
-1.05829506364875));
#16942=CARTESIAN_POINT('Ctrl Pts',(-0.354166711873529,-0.290879136862659,
-1.06688848765783));
#16943=CARTESIAN_POINT('Ctrl Pts',(-0.302426893214944,-0.305251990234488,
-1.08269251410343));
#16944=CARTESIAN_POINT('Ctrl Pts',(-0.275287440920027,-0.308638795020976,
-1.0898803575765));
#16945=CARTESIAN_POINT('Ctrl Pts',(-0.224855950742601,-0.308638795020976,
-1.10139101611326));
#16946=CARTESIAN_POINT('Ctrl Pts',(-0.19728546073067,-0.305251990234488,
-1.10669035995599));
#16947=CARTESIAN_POINT('Ctrl Pts',(-0.143812384801039,-0.290879136862659,
-1.11490049012186));
#16948=CARTESIAN_POINT('Ctrl Pts',(-0.117914228755037,-0.279889827963178,
-1.1178344036749));
#16949=CARTESIAN_POINT('Ctrl Pts',(-0.0680399972366989,-0.251265615809407,
-1.12208997038458));
#16950=CARTESIAN_POINT('Ctrl Pts',(-0.0383992541984084,-0.227269801620063,
-1.12335509974011));
#16951=CARTESIAN_POINT('Ctrl Pts',(0.00639229239215326,-0.177024326825049,
-1.12404235695137));
#16952=CARTESIAN_POINT('Ctrl Pts',(0.0269302585198977,-0.144299303100741,
-1.12357162229597));
#16953=CARTESIAN_POINT('Ctrl Pts',(0.04670325263426,-0.0928409665394228,
-1.12285816383385));
#16954=CARTESIAN_POINT('Ctrl Pts',(0.0515094706813703,-0.0762225747374255,
-1.12263591311425));
#16955=CARTESIAN_POINT('Ctrl Pts',(0.0548532617164176,-0.0595300000000001,
-1.12247250791414));
#16956=CARTESIAN_POINT('',(0.437601487681057,-0.05953,-1.03511272300331));
#16957=CARTESIAN_POINT('Origin',(0.,-0.05953,0.));
#16958=CARTESIAN_POINT('',(0.911784794170997,-0.05953,-0.656964154625313));
#16959=CARTESIAN_POINT('Ctrl Pts',(0.437601487681056,-0.0595300000000001,
-1.03511272300331));
#16960=CARTESIAN_POINT('Ctrl Pts',(0.440685038163619,-0.0762225747374255,
-1.03380912944435));
#16961=CARTESIAN_POINT('Ctrl Pts',(0.445111721969657,-0.0928409665394228,
-1.03192403056628));
#16962=CARTESIAN_POINT('Ctrl Pts',(0.463236132117164,-0.144299303100741,
-1.0239876538093));
#16963=CARTESIAN_POINT('Ctrl Pts',(0.481944444320713,-0.177024326825049,
-1.01550068154148));
#16964=CARTESIAN_POINT('Ctrl Pts',(0.522002043615455,-0.227269801620064,
-0.995447160474328));
#16965=CARTESIAN_POINT('Ctrl Pts',(0.548158511259203,-0.251265615809407,
-0.981446681891443));
#16966=CARTESIAN_POINT('Ctrl Pts',(0.591247219971725,-0.279889827963178,
-0.955972930713954));
#16967=CARTESIAN_POINT('Ctrl Pts',(0.613307674922609,-0.290879136862659,
-0.942092777160053));
#16968=CARTESIAN_POINT('Ctrl Pts',(0.657923009631182,-0.305251990234487,
-0.91149460735272));
#16969=CARTESIAN_POINT('Ctrl Pts',(0.680463863683393,-0.308638795020976,
-0.894757676234429));
#16970=CARTESIAN_POINT('Ctrl Pts',(0.720906778729542,-0.308638795020976,
-0.862505527716294));
#16971=CARTESIAN_POINT('Ctrl Pts',(0.742239891936899,-0.305251990234488,
-0.844254137480381));
#16972=CARTESIAN_POINT('Ctrl Pts',(0.781998747691872,-0.290879136862659,
-0.80756613568454));
#16973=CARTESIAN_POINT('Ctrl Pts',(0.800439809856112,-0.279889827963178,
-0.789147407129765));
#16974=CARTESIAN_POINT('Ctrl Pts',(0.834863020612702,-0.251265615809407,
-0.752807465209441));
#16975=CARTESIAN_POINT('Ctrl Pts',(0.854332839576145,-0.227269801620064,
-0.73042219438957));
#16976=CARTESIAN_POINT('Ctrl Pts',(0.882797231409153,-0.177024326825049,
-0.695831250979106));
#16977=CARTESIAN_POINT('Ctrl Pts',(0.895234408667242,-0.144299303100741,
-0.679480524217551));
#16978=CARTESIAN_POINT('Ctrl Pts',(0.907004864562642,-0.0928409665394228,
-0.663576540841106));
#16979=CARTESIAN_POINT('Ctrl Pts',(0.909827729890942,-0.0762225747374256,
-0.659680317203144));
#16980=CARTESIAN_POINT('Ctrl Pts',(0.911784794170998,-0.0595300000000001,
-0.656964154625312));
#16981=CARTESIAN_POINT('',(1.08212377959455,-0.05953,-0.303251606722892));
#16982=CARTESIAN_POINT('Origin',(0.,-0.05953,0.));
#16983=CARTESIAN_POINT('',(1.08212377959455,-0.05953,0.303251606722892));
#16984=CARTESIAN_POINT('Ctrl Pts',(1.08212377959455,-0.0595300000000001,
-0.303251606722892));
#16985=CARTESIAN_POINT('Ctrl Pts',(1.0830271513892,-0.0762225747374255,
-0.300028012588062));
#16986=CARTESIAN_POINT('Ctrl Pts',(1.08431331394788,-0.0928409665394228,
-0.2953917518996));
#16987=CARTESIAN_POINT('Ctrl Pts',(1.08940878963422,-0.144299303100741,
-0.276273267473431));
#16988=CARTESIAN_POINT('Ctrl Pts',(1.09443784939331,-0.177024326825049,
-0.256354979351213));
#16989=CARTESIAN_POINT('Ctrl Pts',(1.10373487993589,-0.227269801620064,
-0.212533521233765));
#16990=CARTESIAN_POINT('Ctrl Pts',(1.10909715583869,-0.251265615809407,
-0.183354415742157));
#16991=CARTESIAN_POINT('Ctrl Pts',(1.1160463456491,-0.279889827963178,-0.133783682657561));
#16992=CARTESIAN_POINT('Ctrl Pts',(1.11894887330541,-0.290879136862659,
-0.107881990270302));
#16993=CARTESIAN_POINT('Ctrl Pts',(1.12284346704144,-0.305251990234488,
-0.0539226701638766));
#16994=CARTESIAN_POINT('Ctrl Pts',(1.123812,-0.308638795020976,-0.025864214957475));
#16995=CARTESIAN_POINT('Ctrl Pts',(1.123812,-0.308638795020976,0.025864214957475));
#16996=CARTESIAN_POINT('Ctrl Pts',(1.12284346704144,-0.305251990234488,
0.0539226701638766));
#16997=CARTESIAN_POINT('Ctrl Pts',(1.11894887330541,-0.290879136862659,
0.107881990270302));
#16998=CARTESIAN_POINT('Ctrl Pts',(1.1160463456491,-0.279889827963178,0.133783682657561));
#16999=CARTESIAN_POINT('Ctrl Pts',(1.10909715583869,-0.251265615809407,
0.183354415742157));
#17000=CARTESIAN_POINT('Ctrl Pts',(1.10373487993589,-0.227269801620064,
0.212533521233765));
#17001=CARTESIAN_POINT('Ctrl Pts',(1.09443784939331,-0.177024326825049,
0.256354979351213));
#17002=CARTESIAN_POINT('Ctrl Pts',(1.08940878963422,-0.144299303100741,
0.276273267473431));
#17003=CARTESIAN_POINT('Ctrl Pts',(1.08431331394788,-0.0928409665394228,
0.2953917518996));
#17004=CARTESIAN_POINT('Ctrl Pts',(1.0830271513892,-0.0762225747374255,
0.300028012588062));
#17005=CARTESIAN_POINT('Ctrl Pts',(1.08212377959455,-0.0595300000000001,
0.303251606722892));
#17006=CARTESIAN_POINT('Origin',(0.,-0.05953,0.));
#17007=CARTESIAN_POINT('Origin',(0.,-0.05953,0.));
#17008=CARTESIAN_POINT('',(0.0589974094846122,-0.05953,1.07456964270265));
#17009=CARTESIAN_POINT('Origin',(0.,-0.05953,0.));
#17010=CARTESIAN_POINT('Origin',(-0.244773027351946,-0.05953,1.07242070340001));
#17011=CARTESIAN_POINT('Origin',(-0.244773027351946,0.,1.07242070340001));
#17012=CARTESIAN_POINT('',(-0.519393123750572,-0.05953,0.942555777842682));
#17013=CARTESIAN_POINT('Ctrl Pts',(-0.519393123750572,-0.05953,0.942555777842682));
#17014=CARTESIAN_POINT('Ctrl Pts',(-0.513714466572041,-0.0925528133349865,
0.945684988399766));
#17015=CARTESIAN_POINT('Ctrl Pts',(-0.503136848051455,-0.124911173756694,
0.951483858396181));
#17016=CARTESIAN_POINT('Ctrl Pts',(-0.47593627990192,-0.177924977804098,
0.965323333309091));
#17017=CARTESIAN_POINT('Ctrl Pts',(-0.460931856495794,-0.199697230012983,
0.972669835243841));
#17018=CARTESIAN_POINT('Ctrl Pts',(-0.426157505475872,-0.237895043532788,
0.988400002689705));
#17019=CARTESIAN_POINT('Ctrl Pts',(-0.406380688682952,-0.254319232363049,
0.996771768218699));
#17020=CARTESIAN_POINT('Ctrl Pts',(-0.364750145543744,-0.28018331644634,
1.01272583306292));
#17021=CARTESIAN_POINT('Ctrl Pts',(-0.340838910881557,-0.29104845371857,
1.02112815447116));
#17022=CARTESIAN_POINT('Ctrl Pts',(-0.290495481564827,-0.30527573347708,
1.036574285215));
#17023=CARTESIAN_POINT('Ctrl Pts',(-0.264056468041074,-0.308638795020976,
1.04359501395068));
#17024=CARTESIAN_POINT('Ctrl Pts',(-0.214892249704082,-0.308638795020976,
1.05481642595959));
#17025=CARTESIAN_POINT('Ctrl Pts',(-0.188025341585962,-0.30527573347708,
1.05996242598502));
#17026=CARTESIAN_POINT('Ctrl Pts',(-0.135965654106109,-0.29104845371857,
1.06788913840721));
#17027=CARTESIAN_POINT('Ctrl Pts',(-0.110776745452494,-0.28018331644634,
1.07069360430242));
#17028=CARTESIAN_POINT('Ctrl Pts',(-0.0663467128214646,-0.254319232363049,
1.07438230428002));
#17029=CARTESIAN_POINT('Ctrl Pts',(-0.0448960436540983,-0.237895043532788,
1.07542044338697));
#17030=CARTESIAN_POINT('Ctrl Pts',(-0.00674037211528124,-0.199697230012983,
1.07633607767727));
#17031=CARTESIAN_POINT('Ctrl Pts',(0.00996567398334777,-0.177924977804098,
1.07622728347683));
#17032=CARTESIAN_POINT('Ctrl Pts',(0.0404772621979741,-0.124911173756694,
1.07556023164702));
#17033=CARTESIAN_POINT('Ctrl Pts',(0.0525234025782719,-0.0925528133349865,
1.07492508698591));
#17034=CARTESIAN_POINT('Ctrl Pts',(0.0589974094846124,-0.05953,1.07456964270265));
#17035=CARTESIAN_POINT('Origin',(-0.244773027351946,-0.05953,1.07242070340001));
#17036=CARTESIAN_POINT('Origin',(0.,-0.05953,0.));
#17037=CARTESIAN_POINT('',(-0.803348093619616,-0.05953,0.716109245731214));
#17038=CARTESIAN_POINT('Origin',(0.,-0.05953,0.));
#17039=CARTESIAN_POINT('Origin',(-0.991065754692661,-0.05953,0.477272113029314));
#17040=CARTESIAN_POINT('Origin',(-0.991065754692661,0.,0.477272113029314));
#17041=CARTESIAN_POINT('',(-1.06075609691358,-0.05953,0.181596019242328));
#17042=CARTESIAN_POINT('Ctrl Pts',(-1.06075609691358,-0.05953,0.181596019242328));
#17043=CARTESIAN_POINT('Ctrl Pts',(-1.05966202740332,-0.0925528133349865,
0.187986803072856));
#17044=CARTESIAN_POINT('Ctrl Pts',(-1.05760072925372,-0.124911173756694,
0.199872254546857));
#17045=CARTESIAN_POINT('Ctrl Pts',(-1.05146158959546,-0.177924977804098,
0.22976728653846));
#17046=CARTESIAN_POINT('Ctrl Pts',(-1.04785021111757,-0.199697230012983,
0.246078686169301));
#17047=CARTESIAN_POINT('Ctrl Pts',(-1.03846709802406,-0.237895043532788,
0.283073967563097));
#17048=CARTESIAN_POINT('Ctrl Pts',(-1.03268176429485,-0.254319232363049,
0.303755815985685));
#17049=CARTESIAN_POINT('Ctrl Pts',(-1.01919893537026,-0.28018331644634,
0.346251081972725));
#17050=CARTESIAN_POINT('Ctrl Pts',(-1.01085972381132,-0.29104845371857,
0.370184399726282));
#17051=CARTESIAN_POINT('Ctrl Pts',(-0.99154738033959,-0.30527573347708,
0.419174982698463));
#17052=CARTESIAN_POINT('Ctrl Pts',(-0.980551951791748,-0.308638795020976,
0.444223188605045));
#17053=CARTESIAN_POINT('Ctrl Pts',(-0.958671816228589,-0.308638795020976,
0.489657758261848));
#17054=CARTESIAN_POINT('Ctrl Pts',(-0.945943877838127,-0.30527573347708,
0.51387163140139));
#17055=CARTESIAN_POINT('Ctrl Pts',(-0.91968254693063,-0.29104845371857,
0.559515758398093));
#17056=CARTESIAN_POINT('Ctrl Pts',(-0.906170138993533,-0.28018331644634,
0.580957796077825));
#17057=CARTESIAN_POINT('Ctrl Pts',(-0.8813524085237,-0.254319232363049,
0.617994461173994));
#17058=CARTESIAN_POINT('Ctrl Pts',(-0.868789784891799,-0.237895043532788,
0.635412538795143));
#17059=CARTESIAN_POINT('Ctrl Pts',(-0.845715984518854,-0.199697230012983,
0.66581473268113));
#17060=CARTESIAN_POINT('Ctrl Pts',(-0.835214876415962,-0.177924977804098,
0.678808213394124));
#17061=CARTESIAN_POINT('Ctrl Pts',(-0.815669690204649,-0.124911173756694,
0.702247233627224));
#17062=CARTESIAN_POINT('Ctrl Pts',(-0.807662468433796,-0.0925528133349865,
0.711269279199861));
#17063=CARTESIAN_POINT('Ctrl Pts',(-0.803348093619616,-0.05953,0.716109245731214));
#17064=CARTESIAN_POINT('Origin',(-0.991065754692661,-0.05953,0.477272113029314));
#17065=CARTESIAN_POINT('Origin',(0.,-0.05953,0.));
#17066=CARTESIAN_POINT('',(-1.076188,-0.05953,1.31795018948079E-16));
#17067=CARTESIAN_POINT('Origin',(0.,-0.05953,0.));
#17068=CARTESIAN_POINT('',(-1.06075609691358,-0.05953,-0.181596019242328));
#17069=CARTESIAN_POINT('Origin',(0.,-0.05953,0.));
#17070=CARTESIAN_POINT('Origin',(-0.991065754692661,-0.05953,-0.477272113029314));
#17071=CARTESIAN_POINT('Origin',(-0.991065754692661,0.,-0.477272113029314));
#17072=CARTESIAN_POINT('',(-0.803348093619616,-0.05953,-0.716109245731215));
#17073=CARTESIAN_POINT('Ctrl Pts',(-0.803348093619616,-0.05953,-0.716109245731215));
#17074=CARTESIAN_POINT('Ctrl Pts',(-0.807662468433795,-0.0925528133349865,
-0.711269279199862));
#17075=CARTESIAN_POINT('Ctrl Pts',(-0.815669690204649,-0.124911173756694,
-0.702247233627224));
#17076=CARTESIAN_POINT('Ctrl Pts',(-0.835214876415962,-0.177924977804098,
-0.678808213394124));
#17077=CARTESIAN_POINT('Ctrl Pts',(-0.845715984518854,-0.199697230012983,
-0.66581473268113));
#17078=CARTESIAN_POINT('Ctrl Pts',(-0.868789784891799,-0.237895043532788,
-0.635412538795143));
#17079=CARTESIAN_POINT('Ctrl Pts',(-0.8813524085237,-0.254319232363049,
-0.617994461173994));
#17080=CARTESIAN_POINT('Ctrl Pts',(-0.906170138993533,-0.28018331644634,
-0.580957796077826));
#17081=CARTESIAN_POINT('Ctrl Pts',(-0.91968254693063,-0.29104845371857,
-0.559515758398093));
#17082=CARTESIAN_POINT('Ctrl Pts',(-0.945943877838127,-0.30527573347708,
-0.51387163140139));
#17083=CARTESIAN_POINT('Ctrl Pts',(-0.958671816228589,-0.308638795020976,
-0.489657758261848));
#17084=CARTESIAN_POINT('Ctrl Pts',(-0.980551951791748,-0.308638795020976,
-0.444223188605045));
#17085=CARTESIAN_POINT('Ctrl Pts',(-0.99154738033959,-0.30527573347708,
-0.419174982698463));
#17086=CARTESIAN_POINT('Ctrl Pts',(-1.01085972381132,-0.29104845371857,
-0.370184399726282));
#17087=CARTESIAN_POINT('Ctrl Pts',(-1.01919893537026,-0.28018331644634,
-0.346251081972725));
#17088=CARTESIAN_POINT('Ctrl Pts',(-1.03268176429485,-0.254319232363049,
-0.303755815985685));
#17089=CARTESIAN_POINT('Ctrl Pts',(-1.03846709802406,-0.237895043532788,
-0.283073967563097));
#17090=CARTESIAN_POINT('Ctrl Pts',(-1.04785021111757,-0.199697230012983,
-0.246078686169302));
#17091=CARTESIAN_POINT('Ctrl Pts',(-1.05146158959546,-0.177924977804098,
-0.229767286538461));
#17092=CARTESIAN_POINT('Ctrl Pts',(-1.05760072925372,-0.124911173756694,
-0.199872254546858));
#17093=CARTESIAN_POINT('Ctrl Pts',(-1.05966202740332,-0.0925528133349864,
-0.187986803072857));
#17094=CARTESIAN_POINT('Ctrl Pts',(-1.06075609691358,-0.05953,-0.181596019242328));
#17095=CARTESIAN_POINT('Origin',(-0.991065754692661,-0.05953,-0.477272113029314));
#17096=CARTESIAN_POINT('Origin',(0.,-0.05953,0.));
#17097=CARTESIAN_POINT('',(-0.519393123750572,-0.05953,-0.942555777842682));
#17098=CARTESIAN_POINT('Origin',(0.,-0.05953,0.));
#17099=CARTESIAN_POINT('Origin',(-0.244773027351946,-0.05953,-1.07242070340001));
#17100=CARTESIAN_POINT('Origin',(-0.244773027351946,0.,-1.07242070340001));
#17101=CARTESIAN_POINT('',(0.0589974094846125,-0.05953,-1.07456964270265));
#17102=CARTESIAN_POINT('Ctrl Pts',(0.0589974094846127,-0.05953,-1.07456964270265));
#17103=CARTESIAN_POINT('Ctrl Pts',(0.0525234025782722,-0.0925528133349865,
-1.07492508698591));
#17104=CARTESIAN_POINT('Ctrl Pts',(0.0404772621979744,-0.124911173756694,
-1.07556023164702));
#17105=CARTESIAN_POINT('Ctrl Pts',(0.0099656739833481,-0.177924977804098,
-1.07622728347683));
#17106=CARTESIAN_POINT('Ctrl Pts',(-0.00674037211528096,-0.199697230012983,
-1.07633607767727));
#17107=CARTESIAN_POINT('Ctrl Pts',(-0.044896043654098,-0.237895043532788,
-1.07542044338697));
#17108=CARTESIAN_POINT('Ctrl Pts',(-0.0663467128214644,-0.254319232363049,
-1.07438230428002));
#17109=CARTESIAN_POINT('Ctrl Pts',(-0.110776745452493,-0.28018331644634,
-1.07069360430242));
#17110=CARTESIAN_POINT('Ctrl Pts',(-0.135965654106109,-0.29104845371857,
-1.06788913840721));
#17111=CARTESIAN_POINT('Ctrl Pts',(-0.188025341585962,-0.30527573347708,
-1.05996242598502));
#17112=CARTESIAN_POINT('Ctrl Pts',(-0.214892249704082,-0.308638795020976,
-1.05481642595959));
#17113=CARTESIAN_POINT('Ctrl Pts',(-0.264056468041074,-0.308638795020976,
-1.04359501395068));
#17114=CARTESIAN_POINT('Ctrl Pts',(-0.290495481564827,-0.30527573347708,
-1.036574285215));
#17115=CARTESIAN_POINT('Ctrl Pts',(-0.340838910881557,-0.291048453718569,
-1.02112815447116));
#17116=CARTESIAN_POINT('Ctrl Pts',(-0.364750145543744,-0.28018331644634,
-1.01272583306292));
#17117=CARTESIAN_POINT('Ctrl Pts',(-0.406380688682952,-0.254319232363049,
-0.996771768218699));
#17118=CARTESIAN_POINT('Ctrl Pts',(-0.426157505475872,-0.237895043532788,
-0.988400002689705));
#17119=CARTESIAN_POINT('Ctrl Pts',(-0.460931856495794,-0.199697230012983,
-0.972669835243841));
#17120=CARTESIAN_POINT('Ctrl Pts',(-0.475936279901919,-0.177924977804098,
-0.965323333309091));
#17121=CARTESIAN_POINT('Ctrl Pts',(-0.503136848051454,-0.124911173756694,
-0.951483858396181));
#17122=CARTESIAN_POINT('Ctrl Pts',(-0.513714466572041,-0.0925528133349865,
-0.945684988399766));
#17123=CARTESIAN_POINT('Ctrl Pts',(-0.519393123750572,-0.05953,-0.942555777842682));
#17124=CARTESIAN_POINT('Origin',(-0.244773027351946,-0.05953,-1.07242070340001));
#17125=CARTESIAN_POINT('Origin',(0.,-0.05953,0.));
#17126=CARTESIAN_POINT('',(0.413083465285518,-0.05953,-0.993751811093549));
#17127=CARTESIAN_POINT('Origin',(0.,-0.05953,0.));
#17128=CARTESIAN_POINT('Origin',(0.685838782044607,-0.05953,-0.860014630714833));
#17129=CARTESIAN_POINT('Origin',(0.685838782044607,0.,-0.860014630714833));
#17130=CARTESIAN_POINT('',(0.876916659919095,-0.05953,-0.623857181492959));
#17131=CARTESIAN_POINT('Ctrl Pts',(0.876916659919095,-0.05953,-0.623857181492958));
#17132=CARTESIAN_POINT('Ctrl Pts',(0.873158080166742,-0.0925528133349865,
-0.62914037979579));
#17133=CARTESIAN_POINT('Ctrl Pts',(0.866144010579847,-0.124911173756694,
-0.638954437806245));
#17134=CARTESIAN_POINT('Ctrl Pts',(0.847641868610495,-0.177924977804098,
-0.663225258065736));
#17135=CARTESIAN_POINT('Ctrl Pts',(0.837310877969633,-0.199697230012983,
-0.676354402927683));
#17136=CARTESIAN_POINT('Ctrl Pts',(0.81280533416753,-0.237895043532788,
-0.705614819529209));
#17137=CARTESIAN_POINT('Ctrl Pts',(0.798619410861634,-0.254319232363049,
-0.721738358858166));
#17138=CARTESIAN_POINT('Ctrl Pts',(0.768033796848072,-0.28018331644634,
-0.754175290318038));
#17139=CARTESIAN_POINT('Ctrl Pts',(0.750136149454208,-0.29104845371857,
-0.772120216227122));
#17140=CARTESIAN_POINT('Ctrl Pts',(0.711480111898423,-0.30527573347708,
-0.807879894508811));
#17141=CARTESIAN_POINT('Ctrl Pts',(0.690705563850638,-0.308638795020976,
-0.825676810575913));
#17142=CARTESIAN_POINT('Ctrl Pts',(0.651278921914856,-0.308638795020976,
-0.857118508332695));
#17143=CARTESIAN_POINT('Ctrl Pts',(0.629305439856167,-0.30527573347708,
-0.873412008702649));
#17144=CARTESIAN_POINT('Ctrl Pts',(0.585840553788742,-0.29104845371857,
-0.903141581680914));
#17145=CARTESIAN_POINT('Ctrl Pts',(0.564362943424239,-0.28018331644634,
-0.916597376014514));
#17146=CARTESIAN_POINT('Ctrl Pts',(0.525933334162556,-0.254319232363049,
-0.939198248544427));
#17147=CARTESIAN_POINT('Ctrl Pts',(0.507057380724533,-0.237895043532788,
-0.949440676105255));
#17148=CARTESIAN_POINT('Ctrl Pts',(0.473077587363686,-0.199697230012983,
-0.966820759530997));
#17149=CARTESIAN_POINT('Ctrl Pts',(0.457978755888596,-0.177924977804098,
-0.973971221090534));
#17150=CARTESIAN_POINT('Ctrl Pts',(0.430199341854858,-0.124911173756694,
-0.986608710139579));
#17151=CARTESIAN_POINT('Ctrl Pts',(0.419070565453384,-0.0925528133349865,
-0.991263089003441));
#17152=CARTESIAN_POINT('Ctrl Pts',(0.413083465285518,-0.05953,-0.993751811093549));
#17153=CARTESIAN_POINT('Origin',(0.685838782044607,-0.05953,-0.860014630714833));
#17154=CARTESIAN_POINT('Origin',(0.,-0.208355,0.));
#17155=CARTESIAN_POINT('',(-1.076188,-0.35718,1.31795018948079E-16));
#17156=CARTESIAN_POINT('Origin',(0.,-0.35718,0.));
#17157=CARTESIAN_POINT('',(-1.076188,-0.208355,1.31795018948079E-16));
#17158=CARTESIAN_POINT('',(1.03449977959455,-0.05953,0.296632461748266));
#17159=CARTESIAN_POINT('Origin',(0.,-0.05953,0.));
#17160=CARTESIAN_POINT('',(1.03449977959455,-0.05953,-0.296632461748266));
#17161=CARTESIAN_POINT('Ctrl Pts',(1.03449977959455,-0.05953,0.296632461748267));
#17162=CARTESIAN_POINT('Ctrl Pts',(1.03628691421076,-0.0925528133349865,
0.290399865505497));
#17163=CARTESIAN_POINT('Ctrl Pts',(1.03958665287714,-0.124911173756694,
0.278797079997872));
#17164=CARTESIAN_POINT('Ctrl Pts',(1.0470264474309,-0.177924977804098,0.249198913998601));
#17165=CARTESIAN_POINT('Ctrl Pts',(1.05084995891418,-0.199697230012983,
0.232935932341942));
#17166=CARTESIAN_POINT('Ctrl Pts',(1.05844771715377,-0.237895043532788,
0.195533155353269));
#17167=CARTESIAN_POINT('Ctrl Pts',(1.06220882929878,-0.254319232363049,
0.17438929156337));
#17168=CARTESIAN_POINT('Ctrl Pts',(1.06849922508772,-0.28018331644634,0.130252399648131));
#17169=CARTESIAN_POINT('Ctrl Pts',(1.07137013248666,-0.29104845371857,0.105070977154072));
#17170=CARTESIAN_POINT('Ctrl Pts',(1.07522652957392,-0.30527573347708,0.0525526752791107));
#17171=CARTESIAN_POINT('Ctrl Pts',(1.076188,-0.308638795020976,0.025214283908933));
#17172=CARTESIAN_POINT('Ctrl Pts',(1.076188,-0.308638795020976,-0.025214283908933));
#17173=CARTESIAN_POINT('Ctrl Pts',(1.07522652957392,-0.30527573347708,-0.0525526752791107));
#17174=CARTESIAN_POINT('Ctrl Pts',(1.07137013248666,-0.29104845371857,-0.105070977154072));
#17175=CARTESIAN_POINT('Ctrl Pts',(1.06849922508772,-0.28018331644634,-0.130252399648131));
#17176=CARTESIAN_POINT('Ctrl Pts',(1.06220882929878,-0.254319232363049,
-0.17438929156337));
#17177=CARTESIAN_POINT('Ctrl Pts',(1.05844771715377,-0.237895043532788,
-0.195533155353269));
#17178=CARTESIAN_POINT('Ctrl Pts',(1.05084995891418,-0.199697230012983,
-0.232935932341942));
#17179=CARTESIAN_POINT('Ctrl Pts',(1.0470264474309,-0.177924977804098,-0.249198913998601));
#17180=CARTESIAN_POINT('Ctrl Pts',(1.03958665287714,-0.124911173756694,
-0.278797079997872));
#17181=CARTESIAN_POINT('Ctrl Pts',(1.03628691421076,-0.0925528133349865,
-0.290399865505497));
#17182=CARTESIAN_POINT('Ctrl Pts',(1.03449977959455,-0.05953,-0.296632461748267));
#17183=CARTESIAN_POINT('Origin',(0.,-0.05953,0.));
#17184=CARTESIAN_POINT('Origin',(0.,-0.05953,0.));
#17185=CARTESIAN_POINT('Origin',(1.1,-0.05953,0.));
#17186=CARTESIAN_POINT('Origin',(1.1,0.,0.));
#17187=CARTESIAN_POINT('Origin',(1.1,-0.05953,0.));
#17188=CARTESIAN_POINT('Origin',(0.,-0.35718,0.));
#17189=CARTESIAN_POINT('Origin',(0.,-0.05953,0.));
#53829=UNCERTAINTY_MEASURE_WITH_UNIT(LENGTH_MEASURE(0.001),#53910,
'DISTANCE_ACCURACY_VALUE',
'Maximum model space distance between geometric entities at asserted c
onnectivities');
#53859=UNCERTAINTY_MEASURE_WITH_UNIT(LENGTH_MEASURE(0.001),#53910,
'DISTANCE_ACCURACY_VALUE',
'Maximum model space distance between geometric entities at asserted c
onnectivities');
#53879=(
GEOMETRIC_REPRESENTATION_CONTEXT(3)
GLOBAL_UNCERTAINTY_ASSIGNED_CONTEXT((#53829))
GLOBAL_UNIT_ASSIGNED_CONTEXT((#53910,#53912,#53913))
REPRESENTATION_CONTEXT('','3D')
);
#53909=(
GEOMETRIC_REPRESENTATION_CONTEXT(3)
GLOBAL_UNCERTAINTY_ASSIGNED_CONTEXT((#53859))
GLOBAL_UNIT_ASSIGNED_CONTEXT((#53910,#53912,#53913))
REPRESENTATION_CONTEXT('','3D')
);
#53910=(
LENGTH_UNIT()
NAMED_UNIT(*)
SI_UNIT(.CENTI.,.METRE.)
);
#53912=(
NAMED_UNIT(*)
PLANE_ANGLE_UNIT()
SI_UNIT($,.RADIAN.)
);
#53913=(
NAMED_UNIT(*)
SI_UNIT($,.STERADIAN.)
SOLID_ANGLE_UNIT()
);
#53933=SHAPE_DEFINITION_REPRESENTATION(#53982,#54105);
#53982=PRODUCT_DEFINITION_SHAPE('',$,#54155);
#54105=SHAPE_REPRESENTATION('',(#12209),#53879);
#54135=PRODUCT_DEFINITION_CONTEXT('part definition',#54284,'design');
#54155=PRODUCT_DEFINITION('Cage','Cage',#54204,#54135);
#54204=PRODUCT_DEFINITION_FORMATION('',$,#54305);
#54284=APPLICATION_CONTEXT(
'Core Data for Automotive Mechanical Design Process');
#54285=PRODUCT_CONTEXT('part definition',#54284,'mechanical');
#54305=PRODUCT('Cage','Cage','Cage',(#54285));
#54391=COLOUR_RGB('Grey',0.48,0.52,0.57);
#54392=FILL_AREA_STYLE_COLOUR('',#54391);
#54393=FILL_AREA_STYLE('',(#54392));
#54394=SURFACE_STYLE_FILL_AREA(#54393);
#54395=SURFACE_SIDE_STYLE('',(#54394));
#54396=SURFACE_STYLE_USAGE(.BOTH.,#54395);
#54397=PRESENTATION_STYLE_ASSIGNMENT((#54396));
ENDSEC;
END-ISO-10303-21;
